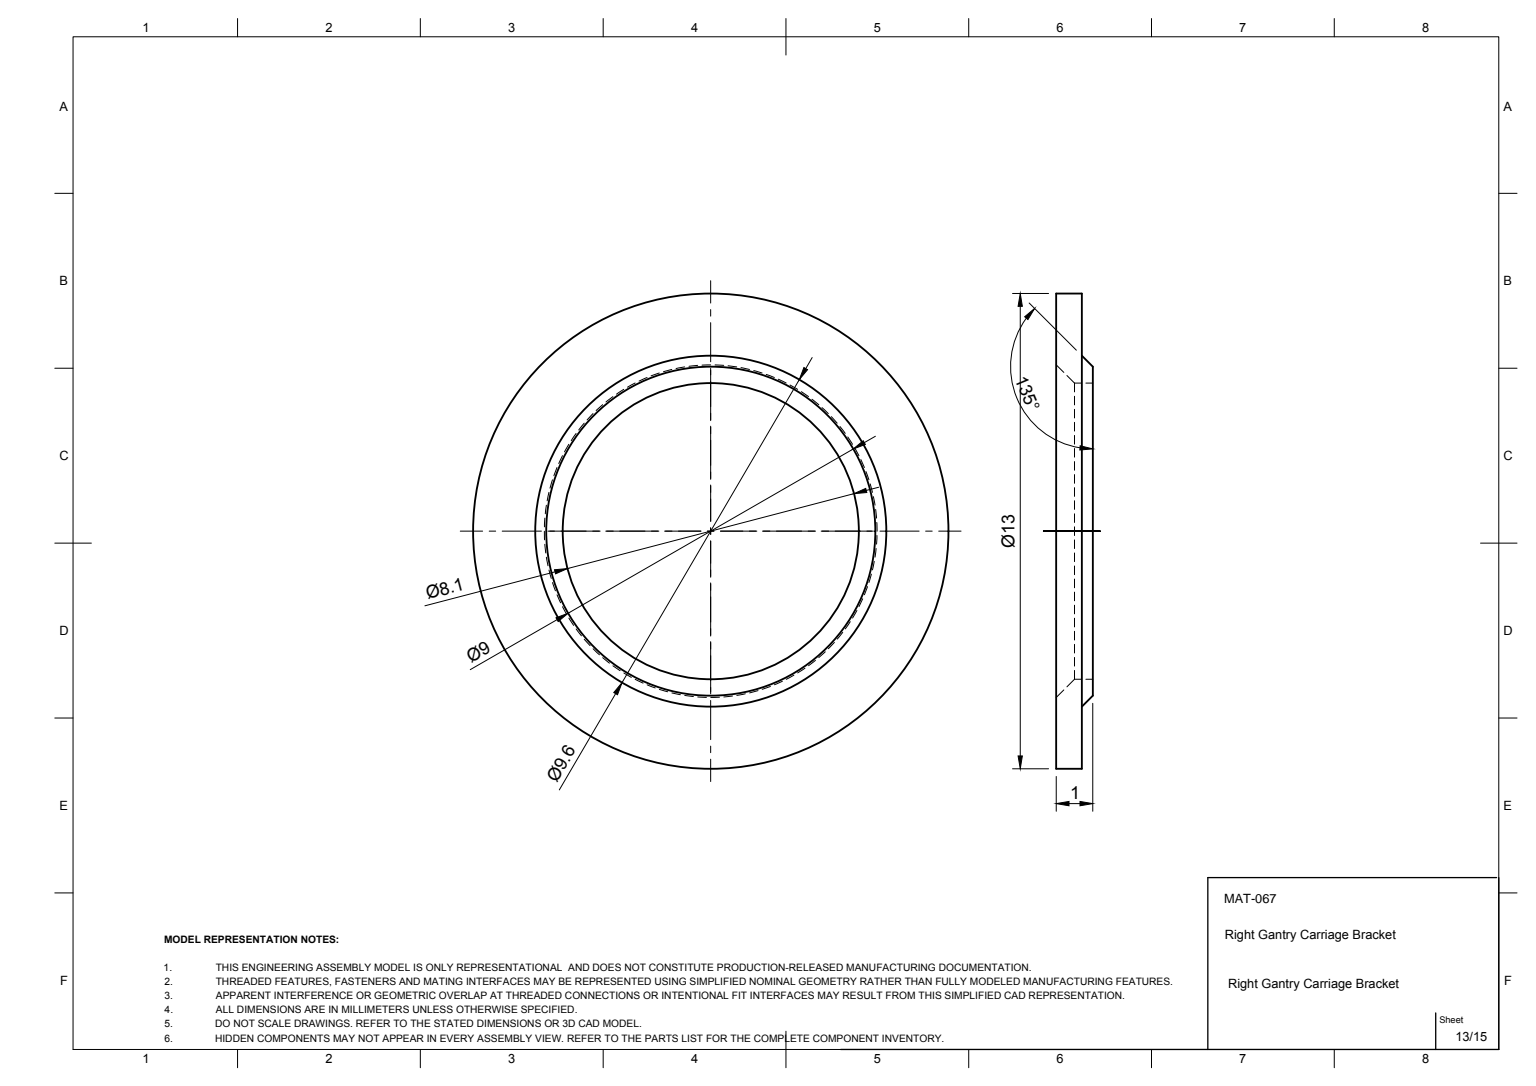
ISO-10303-21;
HEADER;
/* Generated by software containing ST-Developer
 * from STEP Tools, Inc. (www.steptools.com) 
 */

FILE_DESCRIPTION(
/* description */ ('CAx-IF Rec.Pracs.---Representation and Presentation of Product Manufa
cturing Information (PMI)---4.0---2014-10-13'),
/* implementation_level */ '2;1');

FILE_NAME(
/* name */ 'Right Gantry Carriage Bracket.step',
/* time_stamp */ '2026-10-24T16:02:03-07:00',
/* author */ (''),
/* organization */ (''),
/* preprocessor_version */ 'ST-DEVELOPER v20.2',
/* originating_system */ 'Autodesk Translation Framework v15.17.0.0',
/* authorisation */ '');

FILE_SCHEMA (('AP242_MANAGED_MODEL_BASED_3D_ENGINEERING_MIM_LF { 1 0 10303 442 2 1 4 }'));
ENDSEC;

DATA;
#10=MECHANICAL_DESIGN_GEOMETRIC_PRESENTATION_REPRESENTATION('',(#357),#6348);
#321=CONICAL_SURFACE('',#3873,0.0043,0.785398163397448);
#322=CONICAL_SURFACE('',#3879,0.0046499998960644,0.785398163397448);
#335=SHAPE_REPRESENTATION_RELATIONSHIP('SRR','None',#6497,#346);
#346=ADVANCED_BREP_SHAPE_REPRESENTATION('',(#368),#6345);
#357=STYLED_ITEM('',(#6604),#368);
#368=MANIFOLD_SOLID_BREP('Body1',#3396);
#458=CYLINDRICAL_SURFACE('',#3869,0.0065);
#459=CYLINDRICAL_SURFACE('',#3875,0.00405);
#498=FACE_BOUND('',#1053,.T.);
#499=FACE_BOUND('',#1056,.T.);
#500=FACE_BOUND('',#1060,.T.);
#676=CIRCLE('',#3867,0.00650000000001);
#677=CIRCLE('',#3868,0.00479999989272164);
#678=CIRCLE('',#3870,0.00650000000001);
#679=CIRCLE('',#3872,0.00455000000001);
#680=CIRCLE('',#3874,0.00405000000001);
#681=CIRCLE('',#3876,0.00405000000001);
#682=CIRCLE('',#3878,0.00449999989942716);
#847=FACE_OUTER_BOUND('',#1052,.T.);
#848=FACE_OUTER_BOUND('',#1054,.T.);
#849=FACE_OUTER_BOUND('',#1055,.T.);
#850=FACE_OUTER_BOUND('',#1057,.T.);
#851=FACE_OUTER_BOUND('',#1058,.T.);
#852=FACE_OUTER_BOUND('',#1059,.T.);
#853=FACE_OUTER_BOUND('',#1061,.T.);
#1052=EDGE_LOOP('',(#3081));
#1053=EDGE_LOOP('',(#3082));
#1054=EDGE_LOOP('',(#3083,#3084,#3085,#3086));
#1055=EDGE_LOOP('',(#3087));
#1056=EDGE_LOOP('',(#3088));
#1057=EDGE_LOOP('',(#3089,#3090,#3091,#3092));
#1058=EDGE_LOOP('',(#3093,#3094,#3095,#3096));
#1059=EDGE_LOOP('',(#3097));
#1060=EDGE_LOOP('',(#3098));
#1061=EDGE_LOOP('',(#3099,#3100,#3101,#3102));
#1301=LINE('',#6164,#1534);
#1302=LINE('',#6172,#1535);
#1303=LINE('',#6175,#1536);
#1304=LINE('',#6181,#1537);
#1534=VECTOR('',#4901,0.0065);
#1535=VECTOR('',#4912,0.0043);
#1536=VECTOR('',#4915,0.00405);
#1537=VECTOR('',#4924,0.0046499998960644);
#1814=VERTEX_POINT('',#6158);
#1815=VERTEX_POINT('',#6160);
#1816=VERTEX_POINT('',#6163);
#1817=VERTEX_POINT('',#6167);
#1818=VERTEX_POINT('',#6170);
#1819=VERTEX_POINT('',#6174);
#1820=VERTEX_POINT('',#6178);
#2239=EDGE_CURVE('',#1814,#1814,#676,.T.);
#2240=EDGE_CURVE('',#1815,#1815,#677,.T.);
#2241=EDGE_CURVE('',#1814,#1816,#1301,.T.);
#2242=EDGE_CURVE('',#1816,#1816,#678,.T.);
#2243=EDGE_CURVE('',#1817,#1817,#679,.T.);
#2244=EDGE_CURVE('',#1818,#1818,#680,.T.);
#2245=EDGE_CURVE('',#1818,#1817,#1302,.T.);
#2246=EDGE_CURVE('',#1818,#1819,#1303,.T.);
#2247=EDGE_CURVE('',#1819,#1819,#681,.T.);
#2248=EDGE_CURVE('',#1820,#1820,#682,.T.);
#2249=EDGE_CURVE('',#1815,#1820,#1304,.T.);
#3081=ORIENTED_EDGE('',*,*,#2239,.T.);
#3082=ORIENTED_EDGE('',*,*,#2240,.F.);
#3083=ORIENTED_EDGE('',*,*,#2239,.F.);
#3084=ORIENTED_EDGE('',*,*,#2241,.T.);
#3085=ORIENTED_EDGE('',*,*,#2242,.T.);
#3086=ORIENTED_EDGE('',*,*,#2241,.F.);
#3087=ORIENTED_EDGE('',*,*,#2242,.F.);
#3088=ORIENTED_EDGE('',*,*,#2243,.T.);
#3089=ORIENTED_EDGE('',*,*,#2244,.T.);
#3090=ORIENTED_EDGE('',*,*,#2245,.T.);
#3091=ORIENTED_EDGE('',*,*,#2243,.F.);
#3092=ORIENTED_EDGE('',*,*,#2245,.F.);
#3093=ORIENTED_EDGE('',*,*,#2244,.F.);
#3094=ORIENTED_EDGE('',*,*,#2246,.T.);
#3095=ORIENTED_EDGE('',*,*,#2247,.T.);
#3096=ORIENTED_EDGE('',*,*,#2246,.F.);
#3097=ORIENTED_EDGE('',*,*,#2248,.T.);
#3098=ORIENTED_EDGE('',*,*,#2247,.F.);
#3099=ORIENTED_EDGE('',*,*,#2240,.T.);
#3100=ORIENTED_EDGE('',*,*,#2249,.T.);
#3101=ORIENTED_EDGE('',*,*,#2248,.F.);
#3102=ORIENTED_EDGE('',*,*,#2249,.F.);
#3209=PLANE('',#3866);
#3210=PLANE('',#3871);
#3211=PLANE('',#3877);
#3370=ADVANCED_FACE('',(#847,#498),#3209,.F.);
#3371=ADVANCED_FACE('',(#848),#458,.T.);
#3372=ADVANCED_FACE('',(#849,#499),#3210,.F.);
#3373=ADVANCED_FACE('',(#850),#321,.F.);
#3374=ADVANCED_FACE('',(#851),#459,.F.);
#3375=ADVANCED_FACE('',(#852,#500),#3211,.F.);
#3376=ADVANCED_FACE('',(#853),#322,.T.);
#3396=CLOSED_SHELL('',(#3370,#3371,#3372,#3373,#3374,#3375,#3376));
#3865=AXIS2_PLACEMENT_3D('',#6156,#4891,#4892);
#3866=AXIS2_PLACEMENT_3D('',#6157,#4893,#4894);
#3867=AXIS2_PLACEMENT_3D('',#6159,#4895,#4896);
#3868=AXIS2_PLACEMENT_3D('',#6161,#4897,#4898);
#3869=AXIS2_PLACEMENT_3D('',#6162,#4899,#4900);
#3870=AXIS2_PLACEMENT_3D('',#6165,#4902,#4903);
#3871=AXIS2_PLACEMENT_3D('',#6166,#4904,#4905);
#3872=AXIS2_PLACEMENT_3D('',#6168,#4906,#4907);
#3873=AXIS2_PLACEMENT_3D('',#6169,#4908,#4909);
#3874=AXIS2_PLACEMENT_3D('',#6171,#4910,#4911);
#3875=AXIS2_PLACEMENT_3D('',#6173,#4913,#4914);
#3876=AXIS2_PLACEMENT_3D('',#6176,#4916,#4917);
#3877=AXIS2_PLACEMENT_3D('',#6177,#4918,#4919);
#3878=AXIS2_PLACEMENT_3D('',#6179,#4920,#4921);
#3879=AXIS2_PLACEMENT_3D('',#6180,#4922,#4923);
#4891=DIRECTION('axis',(0.,0.,1.));
#4892=DIRECTION('refdir',(1.,0.,0.));
#4893=DIRECTION('center_axis',(0.,-1.,0.));
#4894=DIRECTION('ref_axis',(1.,0.,0.));
#4895=DIRECTION('center_axis',(0.,1.,0.));
#4896=DIRECTION('ref_axis',(1.,0.,0.));
#4897=DIRECTION('center_axis',(0.,1.,0.));
#4898=DIRECTION('ref_axis',(1.,0.,0.));
#4899=DIRECTION('center_axis',(0.,1.,0.));
#4900=DIRECTION('ref_axis',(0.,0.,1.));
#4901=DIRECTION('',(0.,-1.,0.));
#4902=DIRECTION('center_axis',(0.,1.,0.));
#4903=DIRECTION('ref_axis',(1.,0.,0.));
#4904=DIRECTION('center_axis',(0.,1.,0.));
#4905=DIRECTION('ref_axis',(0.,0.,1.));
#4906=DIRECTION('center_axis',(0.,1.,0.));
#4907=DIRECTION('ref_axis',(1.,0.,0.));
#4908=DIRECTION('center_axis',(0.,-1.,0.));
#4909=DIRECTION('ref_axis',(0.,0.,1.));
#4910=DIRECTION('center_axis',(0.,1.,0.));
#4911=DIRECTION('ref_axis',(1.,0.,0.));
#4912=DIRECTION('',(8.65956056235493E-17,-0.707106781186548,-0.707106781186547));
#4913=DIRECTION('center_axis',(0.,1.,0.));
#4914=DIRECTION('ref_axis',(0.,0.,1.));
#4915=DIRECTION('',(0.,1.,0.));
#4916=DIRECTION('center_axis',(0.,1.,0.));
#4917=DIRECTION('ref_axis',(1.,0.,0.));
#4918=DIRECTION('center_axis',(0.,-1.,0.));
#4919=DIRECTION('ref_axis',(1.,0.,0.));
#4920=DIRECTION('center_axis',(0.,1.,0.));
#4921=DIRECTION('ref_axis',(1.,0.,0.));
#4922=DIRECTION('center_axis',(0.,-1.,0.));
#4923=DIRECTION('ref_axis',(0.,0.,1.));
#4924=DIRECTION('',(-8.65956056235493E-17,0.707106781186548,0.707106781186547));
#6156=CARTESIAN_POINT('',(0.,0.,0.));
#6157=CARTESIAN_POINT('Origin',(0.,0.0116999997384846,0.0065));
#6158=CARTESIAN_POINT('',(-7.9602041944578E-19,0.0116999997384946,-0.0065));
#6159=CARTESIAN_POINT('Origin',(0.,0.0116999997384946,0.));
#6160=CARTESIAN_POINT('',(5.87830450451699E-19,0.0116999997384846,-0.00479999989271167));
#6161=CARTESIAN_POINT('Origin',(0.,0.0116999997384946,0.));
#6162=CARTESIAN_POINT('Origin',(0.,0.0113499997351319,0.));
#6163=CARTESIAN_POINT('',(-7.9602041944578E-19,0.0109999997317891,-0.0065));
#6164=CARTESIAN_POINT('',(-7.9602041944578E-19,0.0113499997351319,-0.0065));
#6165=CARTESIAN_POINT('Origin',(0.,0.0109999997317891,0.));
#6166=CARTESIAN_POINT('Origin',(0.,0.0109999997317791,0.00455));
#6167=CARTESIAN_POINT('',(5.57214293612046E-19,0.0109999997317791,-0.00455));
#6168=CARTESIAN_POINT('Origin',(0.,0.0109999997317891,0.));
#6169=CARTESIAN_POINT('Origin',(0.,0.0112499997317791,0.));
#6170=CARTESIAN_POINT('',(4.95981953654678E-19,0.0114999997317791,-0.00405));
#6171=CARTESIAN_POINT('Origin',(0.,0.0114999997317891,0.));
#6172=CARTESIAN_POINT('',(5.26598123633362E-19,0.0112499997317791,-0.0043));
#6173=CARTESIAN_POINT('Origin',(0.,0.0117499997317791,0.));
#6174=CARTESIAN_POINT('',(-4.95981953654678E-19,0.0119999997317891,-0.00405));
#6175=CARTESIAN_POINT('',(-4.95981953654678E-19,0.0117499997317791,-0.00405));
#6176=CARTESIAN_POINT('Origin',(0.,0.0119999997317891,0.));
#6177=CARTESIAN_POINT('Origin',(0.,0.0119999997317791,0.00449999989941716));
#6178=CARTESIAN_POINT('',(5.51091047298466E-19,0.0119999997317791,-0.00449999989941718));
#6179=CARTESIAN_POINT('Origin',(0.,0.0119999997317891,0.));
#6180=CARTESIAN_POINT('Origin',(0.,0.0118499997351319,0.));
#6181=CARTESIAN_POINT('',(5.69460748875079E-19,0.0118499997351319,-0.0046499998960644));
#6320=UNCERTAINTY_MEASURE_WITH_UNIT(LENGTH_MEASURE(1.E-5),#6349,
'DISTANCE_ACCURACY_VALUE',
'Maximum model space distance between geometric entities at asserted c
onnectivities');
#6323=UNCERTAINTY_MEASURE_WITH_UNIT(LENGTH_MEASURE(1.E-5),#6349,
'DISTANCE_ACCURACY_VALUE',
'Maximum model space distance between geometric entities at asserted c
onnectivities');
#6345=(
GEOMETRIC_REPRESENTATION_CONTEXT(3)
GLOBAL_UNCERTAINTY_ASSIGNED_CONTEXT((#6320))
GLOBAL_UNIT_ASSIGNED_CONTEXT((#6349,#6350,#6351))
REPRESENTATION_CONTEXT('','3D')
);
#6348=(
GEOMETRIC_REPRESENTATION_CONTEXT(3)
GLOBAL_UNCERTAINTY_ASSIGNED_CONTEXT((#6323))
GLOBAL_UNIT_ASSIGNED_CONTEXT((#6349,#6350,#6351))
REPRESENTATION_CONTEXT('','3D')
);
#6349=(
LENGTH_UNIT()
NAMED_UNIT(*)
SI_UNIT($,.METRE.)
);
#6350=(
NAMED_UNIT(*)
PLANE_ANGLE_UNIT()
SI_UNIT($,.RADIAN.)
);
#6351=(
NAMED_UNIT(*)
SI_UNIT($,.STERADIAN.)
SOLID_ANGLE_UNIT()
);
#6373=SHAPE_DEFINITION_REPRESENTATION(#6397,#6497);
#6397=PRODUCT_DEFINITION_SHAPE('',$,#6522);
#6497=SHAPE_REPRESENTATION('',(#3865),#6345);
#6500=PRODUCT_DEFINITION_CONTEXT('part definition',#6574,'design');
#6522=PRODUCT_DEFINITION('Right Gantry Carriage Bracket',
'Right Gantry Carriage Bracket',#6546,#6500);
#6546=PRODUCT_DEFINITION_FORMATION('',$,#6597);
#6574=APPLICATION_CONTEXT('Managed model based 3d engineering');
#6575=PRODUCT_CONTEXT('part definition',#6574,'mechanical');
#6597=PRODUCT('Right Gantry Carriage Bracket',
'Right Gantry Carriage Bracket',
'LEGAL AND USAGE DISCLAIMER: this Data/Model is provided \X2\201C\X0\A
S IS\X2\201D\X0\ for informational and representational only. It is a 
geometric approximation and is NOT engineered, certified, or guarantee
d for dimensional accuracy, exact tolerances, or production-level prec
ision. Vendor disclaims all implied warranties including fitness for a
 particular purpose. DO NOT USE FOR DIRECT PHYSICAL MANUFACTURING, AUT
OMATED PRODUCTION, OR SAFETY-CRITICAL SYSTEMS without independent engi
neering verification and resolution of any design discrepancies.',(#6575));
#6604=PRESENTATION_STYLE_ASSIGNMENT((#6610));
#6610=SURFACE_STYLE_USAGE(.BOTH.,#6616);
#6616=SURFACE_SIDE_STYLE('',(#6622));
#6622=SURFACE_STYLE_FILL_AREA(#6628);
#6628=FILL_AREA_STYLE('Opaque(25,25,25)',(#6634));
#6634=FILL_AREA_STYLE_COLOUR('Opaque(25,25,25)',#6640);
#6640=COLOUR_RGB('Opaque(25,25,25)',0.0980392156862745,0.0980392156862745,
0.0980392156862745);
ENDSEC;
END-ISO-10303-21;
